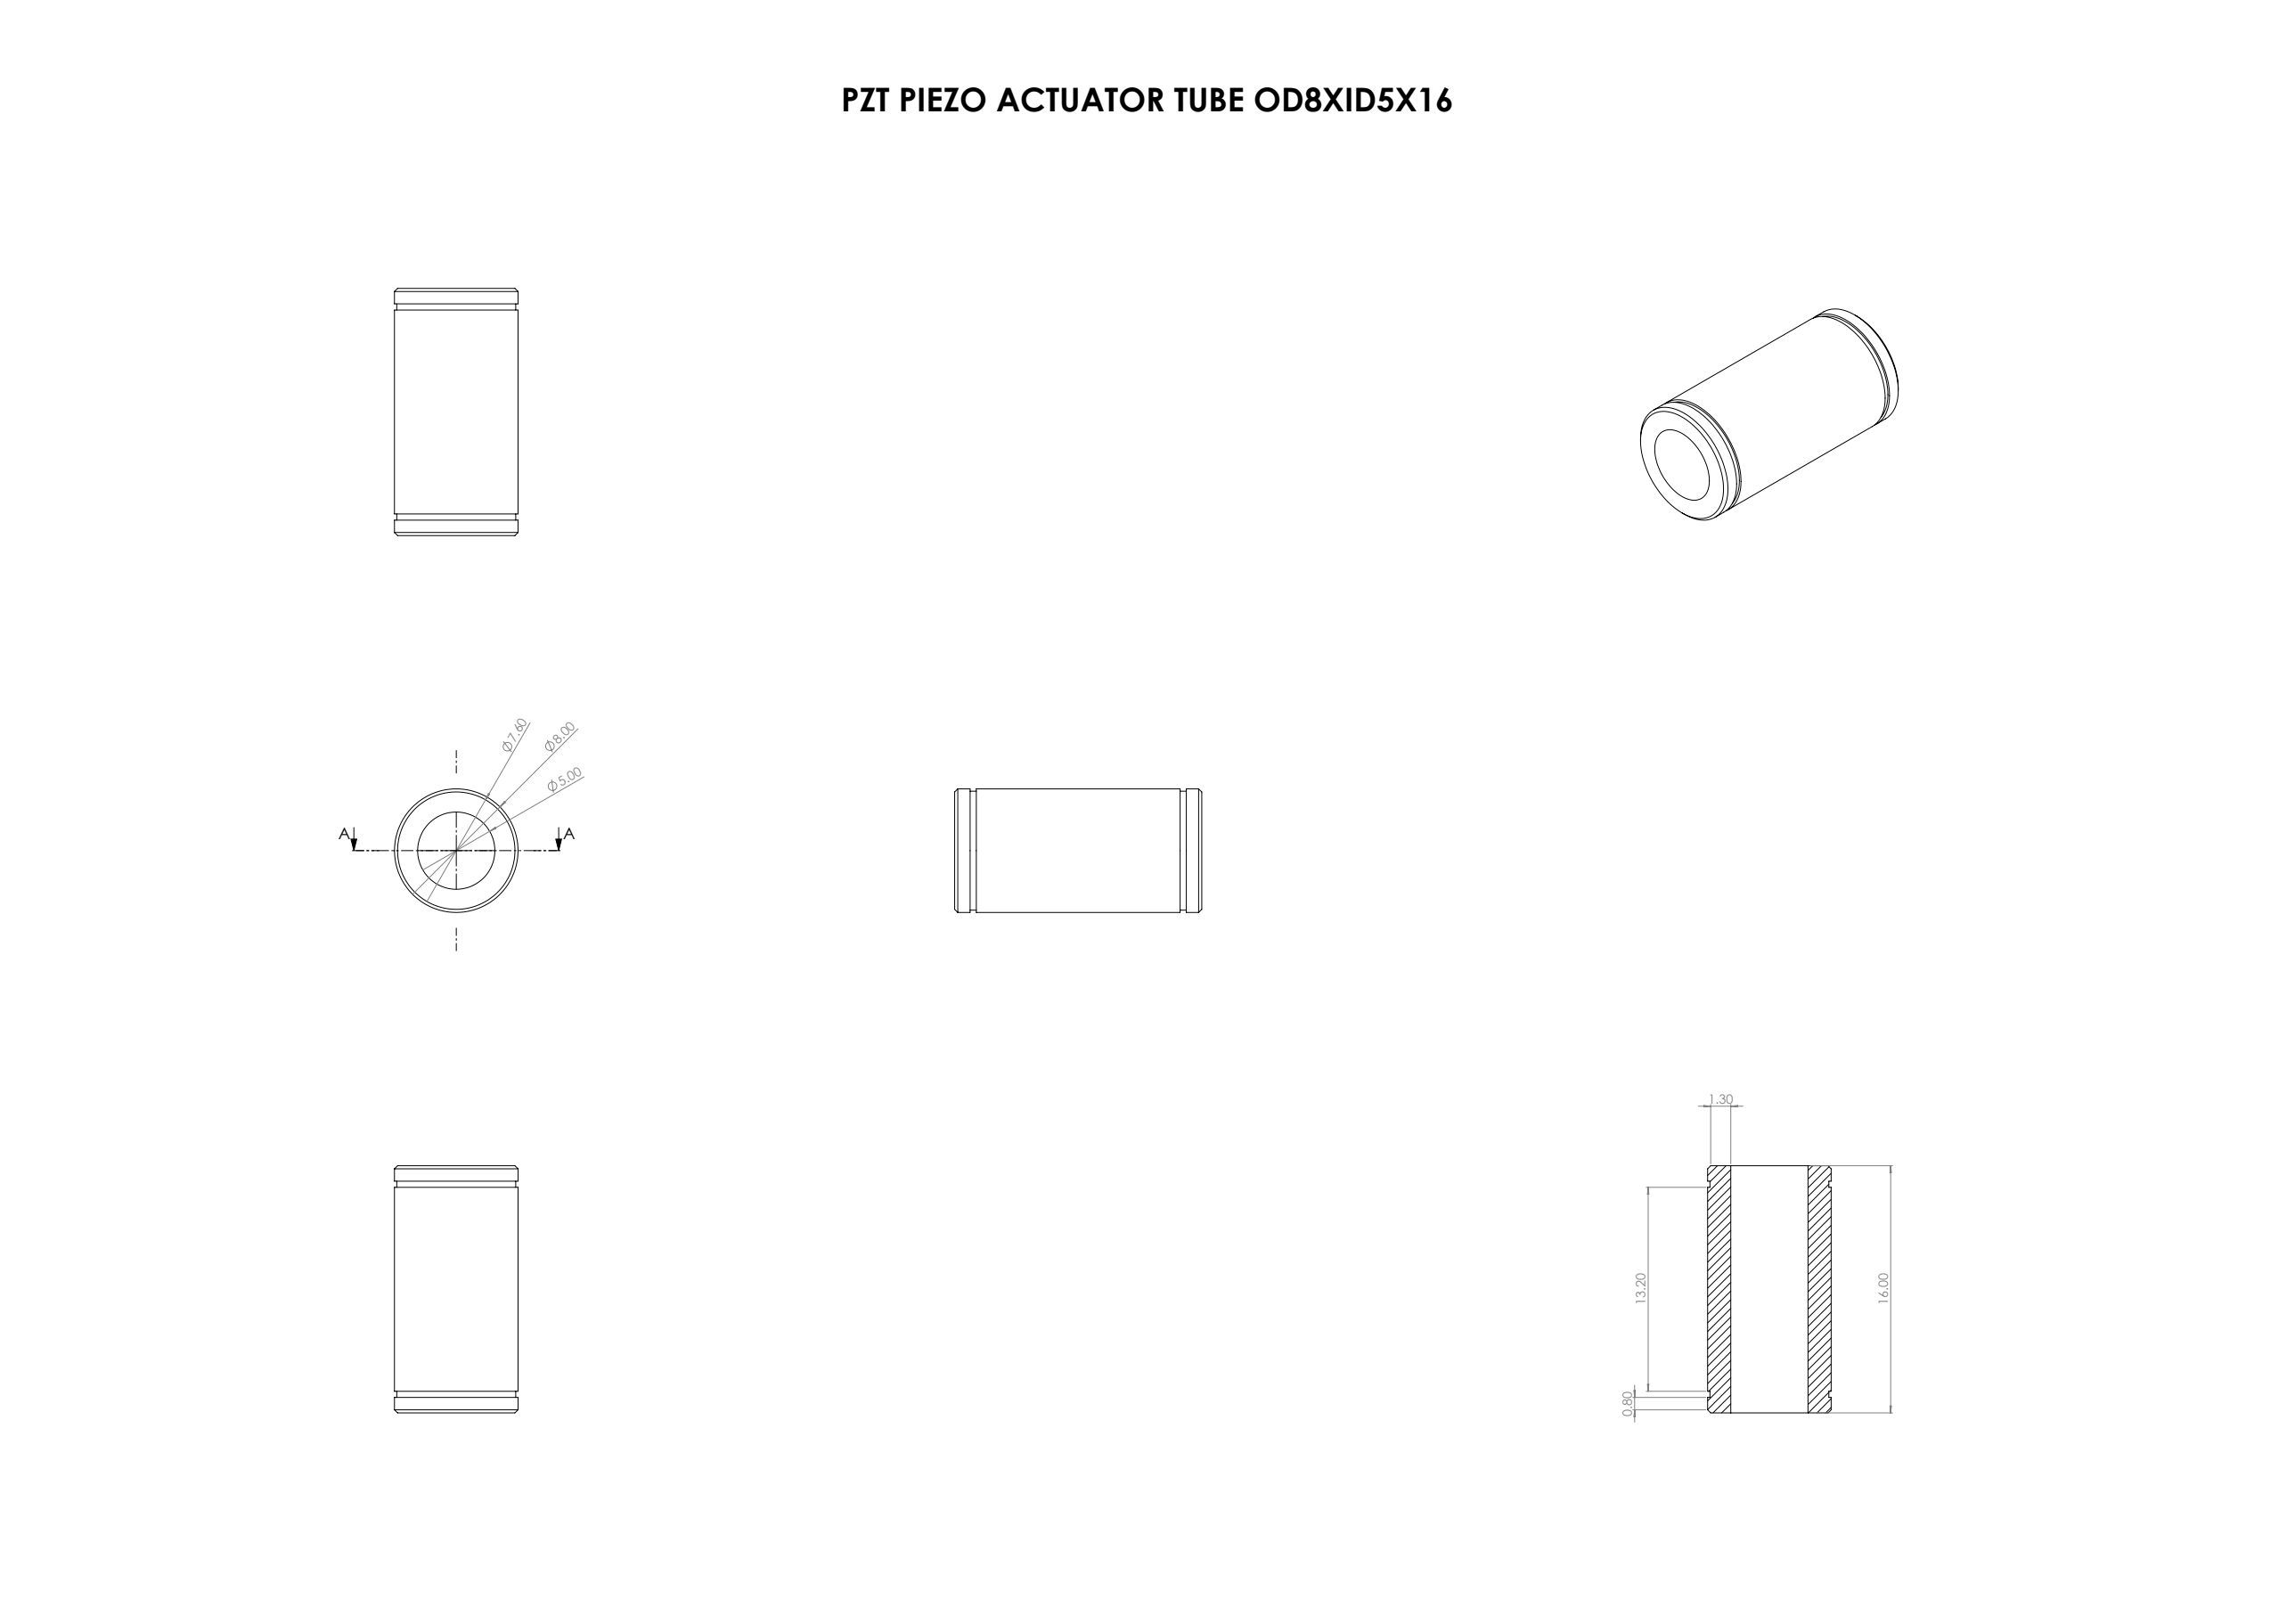
ISO-10303-21;
HEADER;
/* Generated by software containing ST-Developer
 * from STEP Tools, Inc. (www.steptools.com) 
 */

FILE_DESCRIPTION(
/* description */ (''),
/* implementation_level */ '2;1');

FILE_NAME(
/* name */ '06_PZT_Piezo_Actuator_Tube_OD8xID5x16.step',
/* time_stamp */ '2026-10-19T22:59:19-07:00',
/* author */ (''),
/* organization */ (''),
/* preprocessor_version */ 'ST-DEVELOPER v20.2',
/* originating_system */ 'Autodesk Translation Framework v15.15.0.0',
/* authorisation */ '');

FILE_SCHEMA (('AUTOMOTIVE_DESIGN { 1 0 10303 214 3 1 1 }'));
ENDSEC;

DATA;
#10=MECHANICAL_DESIGN_GEOMETRIC_PRESENTATION_REPRESENTATION('',(#918),#53650);
#886=SHAPE_REPRESENTATION_RELATIONSHIP('SRR','None',#53731,#902);
#902=ADVANCED_BREP_SHAPE_REPRESENTATION('',(#934),#53641);
#918=STYLED_ITEM('',(#53951),#934);
#934=MANIFOLD_SOLID_BREP('PZT Tube',#23310);
#1032=CYLINDRICAL_SURFACE('',#24344,0.385);
#1033=CYLINDRICAL_SURFACE('',#24351,0.4);
#1034=CYLINDRICAL_SURFACE('',#24354,0.385);
#1035=CYLINDRICAL_SURFACE('',#24361,0.4);
#1036=CYLINDRICAL_SURFACE('',#24364,0.4);
#1037=CYLINDRICAL_SURFACE('',#24373,0.25);
#1382=FACE_BOUND('',#4146,.T.);
#1383=FACE_BOUND('',#4148,.T.);
#1384=FACE_BOUND('',#4152,.T.);
#1385=FACE_BOUND('',#4154,.T.);
#1386=FACE_BOUND('',#4159,.T.);
#1387=FACE_BOUND('',#4162,.T.);
#1670=PLANE('',#24347);
#1671=PLANE('',#24349);
#1672=PLANE('',#24357);
#1673=PLANE('',#24359);
#1674=PLANE('',#24367);
#1675=PLANE('',#24371);
#2711=FACE_OUTER_BOUND('',#4144,.T.);
#2712=FACE_OUTER_BOUND('',#4145,.T.);
#2713=FACE_OUTER_BOUND('',#4147,.T.);
#2714=FACE_OUTER_BOUND('',#4149,.T.);
#2715=FACE_OUTER_BOUND('',#4150,.T.);
#2716=FACE_OUTER_BOUND('',#4151,.T.);
#2717=FACE_OUTER_BOUND('',#4153,.T.);
#2718=FACE_OUTER_BOUND('',#4155,.T.);
#2719=FACE_OUTER_BOUND('',#4156,.T.);
#2720=FACE_OUTER_BOUND('',#4157,.T.);
#2721=FACE_OUTER_BOUND('',#4158,.T.);
#2722=FACE_OUTER_BOUND('',#4160,.T.);
#2723=FACE_OUTER_BOUND('',#4161,.T.);
#2724=FACE_OUTER_BOUND('',#4163,.T.);
#4144=EDGE_LOOP('',(#17179,#17180,#17181,#17182));
#4145=EDGE_LOOP('',(#17183));
#4146=EDGE_LOOP('',(#17184));
#4147=EDGE_LOOP('',(#17185));
#4148=EDGE_LOOP('',(#17186));
#4149=EDGE_LOOP('',(#17187,#17188,#17189,#17190,#17191));
#4150=EDGE_LOOP('',(#17192,#17193,#17194,#17195));
#4151=EDGE_LOOP('',(#17196));
#4152=EDGE_LOOP('',(#17197));
#4153=EDGE_LOOP('',(#17198));
#4154=EDGE_LOOP('',(#17199));
#4155=EDGE_LOOP('',(#17200,#17201,#17202,#17203));
#4156=EDGE_LOOP('',(#17204,#17205,#17206,#17207,#17208));
#4157=EDGE_LOOP('',(#17209,#17210,#17211,#17212,#17213));
#4158=EDGE_LOOP('',(#17214));
#4159=EDGE_LOOP('',(#17215));
#4160=EDGE_LOOP('',(#17216,#17217,#17218,#17219,#17220));
#4161=EDGE_LOOP('',(#17221));
#4162=EDGE_LOOP('',(#17222));
#4163=EDGE_LOOP('',(#17223,#17224,#17225,#17226));
#5429=CIRCLE('',#24345,0.385);
#5430=CIRCLE('',#24346,0.385);
#5431=CIRCLE('',#24348,0.4);
#5432=CIRCLE('',#24350,0.4);
#5433=CIRCLE('',#24352,0.4);
#5434=CIRCLE('',#24353,0.4);
#5435=CIRCLE('',#24355,0.385);
#5436=CIRCLE('',#24356,0.385);
#5437=CIRCLE('',#24358,0.4);
#5438=CIRCLE('',#24360,0.4);
#5439=CIRCLE('',#24363,0.38);
#5440=CIRCLE('',#24365,0.4);
#5441=CIRCLE('',#24366,0.4);
#5442=CIRCLE('',#24368,0.25);
#5443=CIRCLE('',#24370,0.38);
#5444=CIRCLE('',#24372,0.25);
#6491=LINE('',#35504,#8336);
#6492=LINE('',#35517,#8337);
#6493=LINE('',#35522,#8338);
#6494=LINE('',#35531,#8339);
#6495=LINE('',#35535,#8340);
#6496=LINE('',#35538,#8341);
#6497=LINE('',#35547,#8342);
#6498=LINE('',#35553,#8343);
#8336=VECTOR('',#27993,0.385);
#8337=VECTOR('',#28010,0.4);
#8338=VECTOR('',#28015,0.385);
#8339=VECTOR('',#28028,0.4);
#8340=VECTOR('',#28033,0.39);
#8341=VECTOR('',#28036,0.4);
#8342=VECTOR('',#28047,0.39);
#8343=VECTOR('',#28056,0.25);
#10188=VERTEX_POINT('',#35501);
#10189=VERTEX_POINT('',#35503);
#10190=VERTEX_POINT('',#35507);
#10191=VERTEX_POINT('',#35510);
#10192=VERTEX_POINT('',#35513);
#10193=VERTEX_POINT('',#35514);
#10194=VERTEX_POINT('',#35519);
#10195=VERTEX_POINT('',#35521);
#10196=VERTEX_POINT('',#35525);
#10197=VERTEX_POINT('',#35528);
#10198=VERTEX_POINT('',#35533);
#10199=VERTEX_POINT('',#35537);
#10200=VERTEX_POINT('',#35539);
#10201=VERTEX_POINT('',#35543);
#10202=VERTEX_POINT('',#35546);
#10203=VERTEX_POINT('',#35550);
#12767=EDGE_CURVE('',#10188,#10188,#5429,.T.);
#12768=EDGE_CURVE('',#10188,#10189,#6491,.T.);
#12769=EDGE_CURVE('',#10189,#10189,#5430,.T.);
#12770=EDGE_CURVE('',#10190,#10190,#5431,.T.);
#12771=EDGE_CURVE('',#10191,#10191,#5432,.T.);
#12772=EDGE_CURVE('',#10192,#10193,#5433,.T.);
#12773=EDGE_CURVE('',#10193,#10192,#5434,.T.);
#12774=EDGE_CURVE('',#10193,#10191,#6492,.T.);
#12775=EDGE_CURVE('',#10194,#10194,#5435,.T.);
#12776=EDGE_CURVE('',#10194,#10195,#6493,.T.);
#12777=EDGE_CURVE('',#10195,#10195,#5436,.T.);
#12778=EDGE_CURVE('',#10196,#10196,#5437,.T.);
#12779=EDGE_CURVE('',#10197,#10197,#5438,.T.);
#12780=EDGE_CURVE('',#10190,#10197,#6494,.T.);
#12781=EDGE_CURVE('',#10198,#10198,#5439,.T.);
#12782=EDGE_CURVE('',#10198,#10192,#6495,.T.);
#12783=EDGE_CURVE('',#10196,#10199,#6496,.T.);
#12784=EDGE_CURVE('',#10200,#10199,#5440,.T.);
#12785=EDGE_CURVE('',#10199,#10200,#5441,.T.);
#12786=EDGE_CURVE('',#10201,#10201,#5442,.T.);
#12787=EDGE_CURVE('',#10200,#10202,#6497,.T.);
#12788=EDGE_CURVE('',#10202,#10202,#5443,.T.);
#12789=EDGE_CURVE('',#10203,#10203,#5444,.T.);
#12790=EDGE_CURVE('',#10201,#10203,#6498,.T.);
#17179=ORIENTED_EDGE('',*,*,#12767,.T.);
#17180=ORIENTED_EDGE('',*,*,#12768,.T.);
#17181=ORIENTED_EDGE('',*,*,#12769,.F.);
#17182=ORIENTED_EDGE('',*,*,#12768,.F.);
#17183=ORIENTED_EDGE('',*,*,#12770,.F.);
#17184=ORIENTED_EDGE('',*,*,#12767,.F.);
#17185=ORIENTED_EDGE('',*,*,#12771,.F.);
#17186=ORIENTED_EDGE('',*,*,#12769,.T.);
#17187=ORIENTED_EDGE('',*,*,#12772,.F.);
#17188=ORIENTED_EDGE('',*,*,#12773,.F.);
#17189=ORIENTED_EDGE('',*,*,#12774,.T.);
#17190=ORIENTED_EDGE('',*,*,#12771,.T.);
#17191=ORIENTED_EDGE('',*,*,#12774,.F.);
#17192=ORIENTED_EDGE('',*,*,#12775,.T.);
#17193=ORIENTED_EDGE('',*,*,#12776,.T.);
#17194=ORIENTED_EDGE('',*,*,#12777,.F.);
#17195=ORIENTED_EDGE('',*,*,#12776,.F.);
#17196=ORIENTED_EDGE('',*,*,#12778,.F.);
#17197=ORIENTED_EDGE('',*,*,#12775,.F.);
#17198=ORIENTED_EDGE('',*,*,#12779,.F.);
#17199=ORIENTED_EDGE('',*,*,#12777,.T.);
#17200=ORIENTED_EDGE('',*,*,#12770,.T.);
#17201=ORIENTED_EDGE('',*,*,#12780,.T.);
#17202=ORIENTED_EDGE('',*,*,#12779,.T.);
#17203=ORIENTED_EDGE('',*,*,#12780,.F.);
#17204=ORIENTED_EDGE('',*,*,#12781,.T.);
#17205=ORIENTED_EDGE('',*,*,#12782,.T.);
#17206=ORIENTED_EDGE('',*,*,#12772,.T.);
#17207=ORIENTED_EDGE('',*,*,#12773,.T.);
#17208=ORIENTED_EDGE('',*,*,#12782,.F.);
#17209=ORIENTED_EDGE('',*,*,#12778,.T.);
#17210=ORIENTED_EDGE('',*,*,#12783,.T.);
#17211=ORIENTED_EDGE('',*,*,#12784,.F.);
#17212=ORIENTED_EDGE('',*,*,#12785,.F.);
#17213=ORIENTED_EDGE('',*,*,#12783,.F.);
#17214=ORIENTED_EDGE('',*,*,#12781,.F.);
#17215=ORIENTED_EDGE('',*,*,#12786,.F.);
#17216=ORIENTED_EDGE('',*,*,#12784,.T.);
#17217=ORIENTED_EDGE('',*,*,#12785,.T.);
#17218=ORIENTED_EDGE('',*,*,#12787,.T.);
#17219=ORIENTED_EDGE('',*,*,#12788,.T.);
#17220=ORIENTED_EDGE('',*,*,#12787,.F.);
#17221=ORIENTED_EDGE('',*,*,#12788,.F.);
#17222=ORIENTED_EDGE('',*,*,#12789,.T.);
#17223=ORIENTED_EDGE('',*,*,#12786,.T.);
#17224=ORIENTED_EDGE('',*,*,#12790,.T.);
#17225=ORIENTED_EDGE('',*,*,#12789,.F.);
#17226=ORIENTED_EDGE('',*,*,#12790,.F.);
#21941=CONICAL_SURFACE('',#24362,0.39,0.785398163397448);
#21942=CONICAL_SURFACE('',#24369,0.39,0.785398163397448);
#22450=ADVANCED_FACE('',(#2711),#1032,.T.);
#22451=ADVANCED_FACE('',(#2712,#1382),#1670,.F.);
#22452=ADVANCED_FACE('',(#2713,#1383),#1671,.F.);
#22453=ADVANCED_FACE('',(#2714),#1033,.T.);
#22454=ADVANCED_FACE('',(#2715),#1034,.T.);
#22455=ADVANCED_FACE('',(#2716,#1384),#1672,.F.);
#22456=ADVANCED_FACE('',(#2717,#1385),#1673,.F.);
#22457=ADVANCED_FACE('',(#2718),#1035,.T.);
#22458=ADVANCED_FACE('',(#2719),#21941,.T.);
#22459=ADVANCED_FACE('',(#2720),#1036,.T.);
#22460=ADVANCED_FACE('',(#2721,#1386),#1674,.T.);
#22461=ADVANCED_FACE('',(#2722),#21942,.T.);
#22462=ADVANCED_FACE('',(#2723,#1387),#1675,.T.);
#22463=ADVANCED_FACE('',(#2724),#1037,.F.);
#23310=CLOSED_SHELL('',(#22450,#22451,#22452,#22453,#22454,#22455,#22456,
#22457,#22458,#22459,#22460,#22461,#22462,#22463));
#24343=AXIS2_PLACEMENT_3D('',#35499,#27987,#27988);
#24344=AXIS2_PLACEMENT_3D('',#35500,#27989,#27990);
#24345=AXIS2_PLACEMENT_3D('',#35502,#27991,#27992);
#24346=AXIS2_PLACEMENT_3D('',#35505,#27994,#27995);
#24347=AXIS2_PLACEMENT_3D('',#35506,#27996,#27997);
#24348=AXIS2_PLACEMENT_3D('',#35508,#27998,#27999);
#24349=AXIS2_PLACEMENT_3D('',#35509,#28000,#28001);
#24350=AXIS2_PLACEMENT_3D('',#35511,#28002,#28003);
#24351=AXIS2_PLACEMENT_3D('',#35512,#28004,#28005);
#24352=AXIS2_PLACEMENT_3D('',#35515,#28006,#28007);
#24353=AXIS2_PLACEMENT_3D('',#35516,#28008,#28009);
#24354=AXIS2_PLACEMENT_3D('',#35518,#28011,#28012);
#24355=AXIS2_PLACEMENT_3D('',#35520,#28013,#28014);
#24356=AXIS2_PLACEMENT_3D('',#35523,#28016,#28017);
#24357=AXIS2_PLACEMENT_3D('',#35524,#28018,#28019);
#24358=AXIS2_PLACEMENT_3D('',#35526,#28020,#28021);
#24359=AXIS2_PLACEMENT_3D('',#35527,#28022,#28023);
#24360=AXIS2_PLACEMENT_3D('',#35529,#28024,#28025);
#24361=AXIS2_PLACEMENT_3D('',#35530,#28026,#28027);
#24362=AXIS2_PLACEMENT_3D('',#35532,#28029,#28030);
#24363=AXIS2_PLACEMENT_3D('',#35534,#28031,#28032);
#24364=AXIS2_PLACEMENT_3D('',#35536,#28034,#28035);
#24365=AXIS2_PLACEMENT_3D('',#35540,#28037,#28038);
#24366=AXIS2_PLACEMENT_3D('',#35541,#28039,#28040);
#24367=AXIS2_PLACEMENT_3D('',#35542,#28041,#28042);
#24368=AXIS2_PLACEMENT_3D('',#35544,#28043,#28044);
#24369=AXIS2_PLACEMENT_3D('',#35545,#28045,#28046);
#24370=AXIS2_PLACEMENT_3D('',#35548,#28048,#28049);
#24371=AXIS2_PLACEMENT_3D('',#35549,#28050,#28051);
#24372=AXIS2_PLACEMENT_3D('',#35551,#28052,#28053);
#24373=AXIS2_PLACEMENT_3D('',#35552,#28054,#28055);
#27987=DIRECTION('axis',(0.,0.,1.));
#27988=DIRECTION('refdir',(1.,0.,0.));
#27989=DIRECTION('center_axis',(0.,0.,1.));
#27990=DIRECTION('ref_axis',(1.,0.,0.));
#27991=DIRECTION('center_axis',(0.,0.,1.));
#27992=DIRECTION('ref_axis',(1.,0.,0.));
#27993=DIRECTION('',(0.,0.,1.));
#27994=DIRECTION('center_axis',(0.,0.,1.));
#27995=DIRECTION('ref_axis',(1.,0.,0.));
#27996=DIRECTION('center_axis',(0.,0.,-1.));
#27997=DIRECTION('ref_axis',(-1.,0.,0.));
#27998=DIRECTION('center_axis',(0.,0.,-1.));
#27999=DIRECTION('ref_axis',(1.,0.,0.));
#28000=DIRECTION('center_axis',(0.,0.,1.));
#28001=DIRECTION('ref_axis',(1.,0.,0.));
#28002=DIRECTION('center_axis',(0.,0.,1.));
#28003=DIRECTION('ref_axis',(1.,0.,0.));
#28004=DIRECTION('center_axis',(0.,0.,1.));
#28005=DIRECTION('ref_axis',(1.,0.,0.));
#28006=DIRECTION('center_axis',(0.,0.,1.));
#28007=DIRECTION('ref_axis',(-1.,0.,0.));
#28008=DIRECTION('center_axis',(0.,0.,1.));
#28009=DIRECTION('ref_axis',(-1.,0.,0.));
#28010=DIRECTION('',(0.,0.,-1.));
#28011=DIRECTION('center_axis',(0.,0.,1.));
#28012=DIRECTION('ref_axis',(1.,0.,0.));
#28013=DIRECTION('center_axis',(0.,0.,1.));
#28014=DIRECTION('ref_axis',(1.,0.,0.));
#28015=DIRECTION('',(0.,0.,1.));
#28016=DIRECTION('center_axis',(0.,0.,1.));
#28017=DIRECTION('ref_axis',(1.,0.,0.));
#28018=DIRECTION('center_axis',(0.,0.,-1.));
#28019=DIRECTION('ref_axis',(-1.,0.,0.));
#28020=DIRECTION('center_axis',(0.,0.,-1.));
#28021=DIRECTION('ref_axis',(1.,0.,0.));
#28022=DIRECTION('center_axis',(0.,0.,1.));
#28023=DIRECTION('ref_axis',(1.,0.,0.));
#28024=DIRECTION('center_axis',(0.,0.,1.));
#28025=DIRECTION('ref_axis',(1.,0.,0.));
#28026=DIRECTION('center_axis',(0.,0.,1.));
#28027=DIRECTION('ref_axis',(1.,0.,0.));
#28028=DIRECTION('',(0.,0.,-1.));
#28029=DIRECTION('center_axis',(0.,0.,-1.));
#28030=DIRECTION('ref_axis',(-1.,0.,0.));
#28031=DIRECTION('center_axis',(0.,0.,-1.));
#28032=DIRECTION('ref_axis',(-1.,0.,0.));
#28033=DIRECTION('',(0.707106781186548,8.65956056235493E-17,-0.707106781186548));
#28034=DIRECTION('center_axis',(0.,0.,1.));
#28035=DIRECTION('ref_axis',(1.,0.,0.));
#28036=DIRECTION('',(0.,0.,-1.));
#28037=DIRECTION('center_axis',(0.,0.,-1.));
#28038=DIRECTION('ref_axis',(-1.,0.,0.));
#28039=DIRECTION('center_axis',(0.,0.,-1.));
#28040=DIRECTION('ref_axis',(-1.,0.,0.));
#28041=DIRECTION('center_axis',(0.,0.,1.));
#28042=DIRECTION('ref_axis',(1.,0.,0.));
#28043=DIRECTION('center_axis',(0.,0.,1.));
#28044=DIRECTION('ref_axis',(1.,0.,0.));
#28045=DIRECTION('center_axis',(0.,0.,1.));
#28046=DIRECTION('ref_axis',(-1.,0.,0.));
#28047=DIRECTION('',(-0.707106781186548,-8.65956056235493E-17,-0.707106781186548));
#28048=DIRECTION('center_axis',(0.,0.,1.));
#28049=DIRECTION('ref_axis',(-1.,0.,0.));
#28050=DIRECTION('center_axis',(0.,0.,-1.));
#28051=DIRECTION('ref_axis',(-1.,0.,0.));
#28052=DIRECTION('center_axis',(0.,0.,1.));
#28053=DIRECTION('ref_axis',(1.,0.,0.));
#28054=DIRECTION('center_axis',(0.,0.,1.));
#28055=DIRECTION('ref_axis',(1.,0.,0.));
#28056=DIRECTION('',(0.,0.,-1.));
#35499=CARTESIAN_POINT('',(0.,0.,0.));
#35500=CARTESIAN_POINT('Origin',(0.,0.,1.48));
#35501=CARTESIAN_POINT('',(-0.385,-4.71489017671731E-17,1.46));
#35502=CARTESIAN_POINT('Origin',(0.,0.,1.46));
#35503=CARTESIAN_POINT('',(-0.385,-4.71489017671731E-17,1.5));
#35504=CARTESIAN_POINT('',(-0.385,-4.71489017671731E-17,1.48));
#35505=CARTESIAN_POINT('Origin',(0.,0.,1.5));
#35506=CARTESIAN_POINT('Origin',(0.41,0.,1.46));
#35507=CARTESIAN_POINT('',(-0.4,4.89858719658941E-17,1.46));
#35508=CARTESIAN_POINT('Origin',(0.,0.,1.46));
#35509=CARTESIAN_POINT('Origin',(0.385,0.,1.5));
#35510=CARTESIAN_POINT('',(-0.4,-4.89858719658941E-17,1.5));
#35511=CARTESIAN_POINT('Origin',(0.,0.,1.5));
#35512=CARTESIAN_POINT('Origin',(0.,0.,0.8));
#35513=CARTESIAN_POINT('',(0.4,4.89858719658941E-17,1.58));
#35514=CARTESIAN_POINT('',(-0.4,-4.89858719658941E-17,1.58));
#35515=CARTESIAN_POINT('Origin',(0.,0.,1.58));
#35516=CARTESIAN_POINT('Origin',(0.,0.,1.58));
#35517=CARTESIAN_POINT('',(-0.4,-4.89858719658941E-17,0.8));
#35518=CARTESIAN_POINT('Origin',(0.,0.,0.12));
#35519=CARTESIAN_POINT('',(-0.385,-4.71489017671731E-17,0.1));
#35520=CARTESIAN_POINT('Origin',(0.,0.,0.1));
#35521=CARTESIAN_POINT('',(-0.385,-4.71489017671731E-17,0.14));
#35522=CARTESIAN_POINT('',(-0.385,-4.71489017671731E-17,0.12));
#35523=CARTESIAN_POINT('Origin',(0.,0.,0.14));
#35524=CARTESIAN_POINT('Origin',(0.41,0.,0.1));
#35525=CARTESIAN_POINT('',(-0.4,4.89858719658941E-17,0.1));
#35526=CARTESIAN_POINT('Origin',(0.,0.,0.1));
#35527=CARTESIAN_POINT('Origin',(0.385,0.,0.14));
#35528=CARTESIAN_POINT('',(-0.4,-4.89858719658941E-17,0.14));
#35529=CARTESIAN_POINT('Origin',(0.,0.,0.14));
#35530=CARTESIAN_POINT('Origin',(0.,0.,0.8));
#35531=CARTESIAN_POINT('',(-0.4,-4.89858719658941E-17,0.8));
#35532=CARTESIAN_POINT('Origin',(0.,0.,1.59));
#35533=CARTESIAN_POINT('',(0.38,-4.65365783675994E-17,1.6));
#35534=CARTESIAN_POINT('Origin',(0.,0.,1.6));
#35535=CARTESIAN_POINT('',(0.39,4.77612251667468E-17,1.59));
#35536=CARTESIAN_POINT('Origin',(0.,0.,0.8));
#35537=CARTESIAN_POINT('',(-0.4,-4.89858719658941E-17,0.02));
#35538=CARTESIAN_POINT('',(-0.4,-4.89858719658941E-17,0.8));
#35539=CARTESIAN_POINT('',(0.4,-4.89858719658941E-17,0.02));
#35540=CARTESIAN_POINT('Origin',(0.,0.,0.02));
#35541=CARTESIAN_POINT('Origin',(0.,0.,0.02));
#35542=CARTESIAN_POINT('Origin',(0.25,0.,1.6));
#35543=CARTESIAN_POINT('',(-0.25,-3.06161699786838E-17,1.6));
#35544=CARTESIAN_POINT('Origin',(0.,0.,1.6));
#35545=CARTESIAN_POINT('Origin',(0.,0.,0.01));
#35546=CARTESIAN_POINT('',(0.38,4.65365783675994E-17,0.));
#35547=CARTESIAN_POINT('',(0.39,4.77612251667468E-17,0.01));
#35548=CARTESIAN_POINT('Origin',(0.,0.,0.));
#35549=CARTESIAN_POINT('Origin',(0.4,0.,0.));
#35550=CARTESIAN_POINT('',(-0.25,-3.06161699786838E-17,0.));
#35551=CARTESIAN_POINT('Origin',(0.,0.,0.));
#35552=CARTESIAN_POINT('Origin',(0.,0.,0.8));
#35553=CARTESIAN_POINT('',(-0.25,-3.06161699786838E-17,0.8));
#53623=UNCERTAINTY_MEASURE_WITH_UNIT(LENGTH_MEASURE(0.001),#53651,
'DISTANCE_ACCURACY_VALUE',
'Maximum model space distance between geometric entities at asserted c
onnectivities');
#53632=UNCERTAINTY_MEASURE_WITH_UNIT(LENGTH_MEASURE(0.001),#53651,
'DISTANCE_ACCURACY_VALUE',
'Maximum model space distance between geometric entities at asserted c
onnectivities');
#53641=(
GEOMETRIC_REPRESENTATION_CONTEXT(3)
GLOBAL_UNCERTAINTY_ASSIGNED_CONTEXT((#53623))
GLOBAL_UNIT_ASSIGNED_CONTEXT((#53651,#53653,#53654))
REPRESENTATION_CONTEXT('','3D')
);
#53650=(
GEOMETRIC_REPRESENTATION_CONTEXT(3)
GLOBAL_UNCERTAINTY_ASSIGNED_CONTEXT((#53632))
GLOBAL_UNIT_ASSIGNED_CONTEXT((#53651,#53653,#53654))
REPRESENTATION_CONTEXT('','3D')
);
#53651=(
LENGTH_UNIT()
NAMED_UNIT(*)
SI_UNIT(.CENTI.,.METRE.)
);
#53653=(
NAMED_UNIT(*)
PLANE_ANGLE_UNIT()
SI_UNIT($,.RADIAN.)
);
#53654=(
NAMED_UNIT(*)
SI_UNIT($,.STERADIAN.)
SOLID_ANGLE_UNIT()
);
#53663=SHAPE_DEFINITION_REPRESENTATION(#53680,#53731);
#53680=PRODUCT_DEFINITION_SHAPE('',$,#53749);
#53731=SHAPE_REPRESENTATION('',(#24343),#53641);
#53740=PRODUCT_DEFINITION_CONTEXT('part definition',#53793,'design');
#53749=PRODUCT_DEFINITION('2026-10-18-22-44-40-399',
'06_PZT_Piezo_Actuator_Tube_OD8xID5x16',#53766,#53740);
#53766=PRODUCT_DEFINITION_FORMATION('',$,#53803);
#53793=APPLICATION_CONTEXT(
'Core Data for Automotive Mechanical Design Process');
#53794=PRODUCT_CONTEXT('part definition',#53793,'mechanical');
#53803=PRODUCT('2026-10-18-22-44-40-399',
'06_PZT_Piezo_Actuator_Tube_OD8xID5x16',$,(#53794));
#53945=COLOUR_RGB('Sky Blue',0.24,0.69,0.87);
#53946=FILL_AREA_STYLE_COLOUR('',#53945);
#53947=FILL_AREA_STYLE('',(#53946));
#53948=SURFACE_STYLE_FILL_AREA(#53947);
#53949=SURFACE_SIDE_STYLE('',(#53948));
#53950=SURFACE_STYLE_USAGE(.BOTH.,#53949);
#53951=PRESENTATION_STYLE_ASSIGNMENT((#53950));
ENDSEC;
END-ISO-10303-21;
